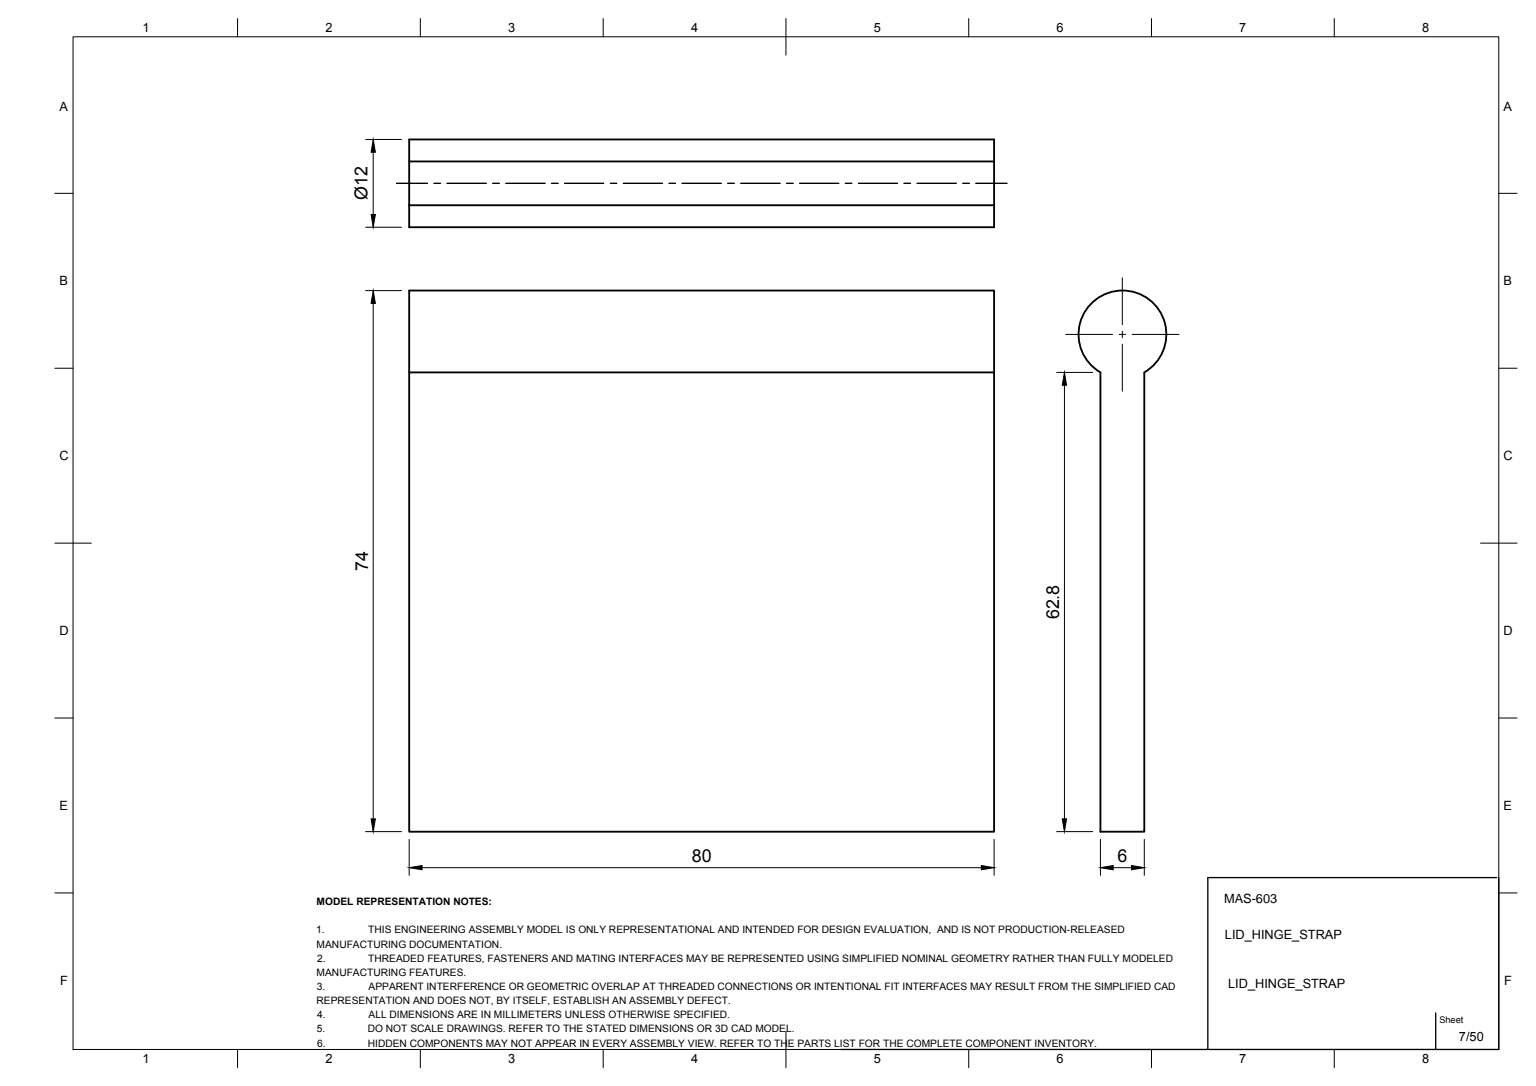
ISO-10303-21;
HEADER;
FILE_DESCRIPTION((''),'2;1');
FILE_NAME('LID_HINGE_STRAP.step','2026-10-01T22:06:14-07:00',(''),(''),'','','');
FILE_SCHEMA (('AUTOMOTIVE_DESIGN { 1 0 10303 214 3 1 1 }'));
ENDSEC;
DATA;
#10=MECHANICAL_DESIGN_GEOMETRIC_PRESENTATION_REPRESENTATION('',(#983),#50440);
#893=SHAPE_REPRESENTATION_RELATIONSHIP('SRR','None',#50623,#938) ;
#938=ADVANCED_BREP_SHAPE_REPRESENTATION('',(#1039),#50392) ;
#983=STYLED_ITEM('',(#50885),#1039) ;
#1039=MANIFOLD_SOLID_BREP('LID_HINGE_STRAP',#28631) ;
#1478=PLANE('',#29331) ;
#1479=PLANE('',#29332) ;
#1480=PLANE('',#29333) ;
#1481=PLANE('',#29334) ;
#1482=PLANE('',#29338) ;
#2419=FACE_OUTER_BOUND('',#3991,.T.) ;
#2420=FACE_OUTER_BOUND('',#3992,.T.) ;
#2421=FACE_OUTER_BOUND('',#3993,.T.) ;
#2422=FACE_OUTER_BOUND('',#3994,.T.) ;
#2423=FACE_OUTER_BOUND('',#3995,.T.) ;
#2424=FACE_OUTER_BOUND('',#3996,.T.) ;
#3991=EDGE_LOOP('',(#18977,#18978,#18979,#18980)) ;
#3992=EDGE_LOOP('',(#18981,#18982,#18983,#18984)) ;
#3993=EDGE_LOOP('',(#18985,#18986,#18987,#18988)) ;
#3994=EDGE_LOOP('',(#18989,#18990,#18991,#18992)) ;
#3995=EDGE_LOOP('',(#18993,#18994,#18995,#18996)) ;
#3996=EDGE_LOOP('',(#18997,#18998,#18999,#19000)) ;
#5885=LINE('',#41663,#8357) ;
#5886=LINE('',#41665,#8358) ;
#5887=LINE('',#41667,#8359) ;
#5888=LINE('',#41668,#8360) ;
#5889=LINE('',#41672,#8361) ;
#5890=LINE('',#41674,#8362) ;
#5891=LINE('',#41676,#8363) ;
#5892=LINE('',#41677,#8364) ;
#5893=LINE('',#41679,#8365) ;
#5894=LINE('',#41680,#8366) ;
#8357=VECTOR('',#32774,1.) ;
#8358=VECTOR('',#32775,1.) ;
#8359=VECTOR('',#32776,1.) ;
#8360=VECTOR('',#32777,1.) ;
#8361=VECTOR('',#32780,1.) ;
#8362=VECTOR('',#32781,1.) ;
#8363=VECTOR('',#32782,1.) ;
#8364=VECTOR('',#32783,1.) ;
#8365=VECTOR('',#32786,1.) ;
#8366=VECTOR('',#32787,1.) ;
#10724=CIRCLE('',#29335,0.6) ;
#10725=CIRCLE('',#29337,0.6) ;
#11983=VERTEX_POINT('',#41661) ;
#11984=VERTEX_POINT('',#41662) ;
#11985=VERTEX_POINT('',#41664) ;
#11986=VERTEX_POINT('',#41666) ;
#11987=VERTEX_POINT('',#41670) ;
#11988=VERTEX_POINT('',#41671) ;
#11989=VERTEX_POINT('',#41673) ;
#11990=VERTEX_POINT('',#41675) ;
#14754=EDGE_CURVE('',#11983,#11984,#5885,.T.) ;
#14755=EDGE_CURVE('',#11983,#11985,#5886,.T.) ;
#14756=EDGE_CURVE('',#11985,#11986,#5887,.T.) ;
#14757=EDGE_CURVE('',#11986,#11984,#5888,.T.) ;
#14758=EDGE_CURVE('',#11987,#11988,#5889,.T.) ;
#14759=EDGE_CURVE('',#11987,#11989,#5890,.T.) ;
#14760=EDGE_CURVE('',#11989,#11990,#5891,.T.) ;
#14761=EDGE_CURVE('',#11990,#11988,#5892,.T.) ;
#14762=EDGE_CURVE('',#11985,#11990,#5893,.T.) ;
#14763=EDGE_CURVE('',#11986,#11989,#5894,.T.) ;
#14764=EDGE_CURVE('',#11987,#11984,#10724,.T.) ;
#14765=EDGE_CURVE('',#11983,#11988,#10725,.T.) ;
#18977=ORIENTED_EDGE('',*,*,#14754,.F.) ;
#18978=ORIENTED_EDGE('',*,*,#14755,.T.) ;
#18979=ORIENTED_EDGE('',*,*,#14756,.T.) ;
#18980=ORIENTED_EDGE('',*,*,#14757,.T.) ;
#18981=ORIENTED_EDGE('',*,*,#14758,.F.) ;
#18982=ORIENTED_EDGE('',*,*,#14759,.T.) ;
#18983=ORIENTED_EDGE('',*,*,#14760,.T.) ;
#18984=ORIENTED_EDGE('',*,*,#14761,.T.) ;
#18985=ORIENTED_EDGE('',*,*,#14762,.T.) ;
#18986=ORIENTED_EDGE('',*,*,#14760,.F.) ;
#18987=ORIENTED_EDGE('',*,*,#14763,.F.) ;
#18988=ORIENTED_EDGE('',*,*,#14756,.F.) ;
#18989=ORIENTED_EDGE('',*,*,#14764,.T.) ;
#18990=ORIENTED_EDGE('',*,*,#14757,.F.) ;
#18991=ORIENTED_EDGE('',*,*,#14763,.T.) ;
#18992=ORIENTED_EDGE('',*,*,#14759,.F.) ;
#18993=ORIENTED_EDGE('',*,*,#14754,.T.) ;
#18994=ORIENTED_EDGE('',*,*,#14764,.F.) ;
#18995=ORIENTED_EDGE('',*,*,#14758,.T.) ;
#18996=ORIENTED_EDGE('',*,*,#14765,.F.) ;
#18997=ORIENTED_EDGE('',*,*,#14765,.T.) ;
#18998=ORIENTED_EDGE('',*,*,#14761,.F.) ;
#18999=ORIENTED_EDGE('',*,*,#14762,.F.) ;
#19000=ORIENTED_EDGE('',*,*,#14755,.F.) ;
#26658=CYLINDRICAL_SURFACE('',#29336,0.6) ;
#27154=ADVANCED_FACE('',(#2419),#1478,.T.) ;
#27155=ADVANCED_FACE('',(#2420),#1479,.F.) ;
#27156=ADVANCED_FACE('',(#2421),#1480,.F.) ;
#27157=ADVANCED_FACE('',(#2422),#1481,.T.) ;
#27158=ADVANCED_FACE('',(#2423),#26658,.T.) ;
#27159=ADVANCED_FACE('',(#2424),#1482,.T.) ;
#28631=CLOSED_SHELL('',(#27154,#27155,#27156,#27157,#27158,#27159)) ;
#29330=AXIS2_PLACEMENT_3D('',#41659,#32770,#32771) ;
#29331=AXIS2_PLACEMENT_3D('',#41660,#32772,#32773) ;
#29332=AXIS2_PLACEMENT_3D('',#41669,#32778,#32779) ;
#29333=AXIS2_PLACEMENT_3D('',#41678,#32784,#32785) ;
#29334=AXIS2_PLACEMENT_3D('',#41681,#32788,#32789) ;
#29335=AXIS2_PLACEMENT_3D('',#41682,#32790,#32791) ;
#29336=AXIS2_PLACEMENT_3D('',#41683,#32792,#32793) ;
#29337=AXIS2_PLACEMENT_3D('',#41684,#32794,#32795) ;
#29338=AXIS2_PLACEMENT_3D('',#41685,#32796,#32797) ;
#32770=DIRECTION('axis',(0.,0.,1.)) ;
#32771=DIRECTION('refdir',(1.,0.,0.)) ;
#32772=DIRECTION('center_axis',(0.,0.,1.)) ;
#32773=DIRECTION('ref_axis',(1.,0.,0.)) ;
#32774=DIRECTION('',(1.,0.,0.)) ;
#32775=DIRECTION('',(0.,-1.,0.)) ;
#32776=DIRECTION('',(1.,0.,0.)) ;
#32777=DIRECTION('',(0.,1.,0.)) ;
#32778=DIRECTION('center_axis',(0.,0.,1.)) ;
#32779=DIRECTION('ref_axis',(1.,0.,0.)) ;
#32780=DIRECTION('',(-1.,0.,0.)) ;
#32781=DIRECTION('',(0.,-1.,0.)) ;
#32782=DIRECTION('',(-1.,0.,0.)) ;
#32783=DIRECTION('',(0.,1.,0.)) ;
#32784=DIRECTION('center_axis',(0.,1.,0.)) ;
#32785=DIRECTION('ref_axis',(0.,0.,1.)) ;
#32786=DIRECTION('',(0.,0.,-1.)) ;
#32787=DIRECTION('',(0.,0.,-1.)) ;
#32788=DIRECTION('center_axis',(1.,0.,0.)) ;
#32789=DIRECTION('ref_axis',(0.,0.,-1.)) ;
#32790=DIRECTION('center_axis',(1.,0.,0.)) ;
#32791=DIRECTION('ref_axis',(0.,0.,-1.)) ;
#32792=DIRECTION('center_axis',(1.,0.,0.)) ;
#32793=DIRECTION('ref_axis',(0.,1.,1.83697019872103E-16)) ;
#32794=DIRECTION('center_axis',(-1.,0.,0.)) ;
#32795=DIRECTION('ref_axis',(0.,0.,-1.)) ;
#32796=DIRECTION('center_axis',(-1.,0.,0.)) ;
#32797=DIRECTION('ref_axis',(0.,0.,1.)) ;
#41659=CARTESIAN_POINT('',(0.,0.,0.)) ;
#41660=CARTESIAN_POINT('Origin',(0.,53.4,112.6)) ;
#41661=CARTESIAN_POINT('',(-4.,56.2803847577293,112.6)) ;
#41662=CARTESIAN_POINT('',(4.,56.2803847577293,112.6)) ;
#41663=CARTESIAN_POINT('',(0.,56.2803847577293,112.6)) ;
#41664=CARTESIAN_POINT('',(-4.,50.,112.6)) ;
#41665=CARTESIAN_POINT('',(-4.,53.4,112.6)) ;
#41666=CARTESIAN_POINT('',(4.,50.,112.6)) ;
#41667=CARTESIAN_POINT('',(0.,50.,112.6)) ;
#41668=CARTESIAN_POINT('',(4.,53.4,112.6)) ;
#41669=CARTESIAN_POINT('Origin',(0.,53.4,112.)) ;
#41670=CARTESIAN_POINT('',(4.,56.2803847577293,112.)) ;
#41671=CARTESIAN_POINT('',(-4.,56.2803847577293,112.)) ;
#41672=CARTESIAN_POINT('',(0.,56.2803847577293,112.)) ;
#41673=CARTESIAN_POINT('',(4.,50.,112.)) ;
#41674=CARTESIAN_POINT('',(4.,53.4,112.)) ;
#41675=CARTESIAN_POINT('',(-4.,50.,112.)) ;
#41676=CARTESIAN_POINT('',(0.,50.,112.)) ;
#41677=CARTESIAN_POINT('',(-4.,53.4,112.)) ;
#41678=CARTESIAN_POINT('Origin',(0.,50.,112.3)) ;
#41679=CARTESIAN_POINT('',(-4.,50.,112.3)) ;
#41680=CARTESIAN_POINT('',(4.,50.,112.3)) ;
#41681=CARTESIAN_POINT('Origin',(4.,56.8,112.3)) ;
#41682=CARTESIAN_POINT('Origin',(4.,56.8,112.3)) ;
#41683=CARTESIAN_POINT('Origin',(0.,56.8,112.3)) ;
#41684=CARTESIAN_POINT('Origin',(-4.,56.8,112.3)) ;
#41685=CARTESIAN_POINT('Origin',(-4.,56.8,112.3)) ;
#50339=UNCERTAINTY_MEASURE_WITH_UNIT(LENGTH_MEASURE(0.001),#50441,
'DISTANCE_ACCURACY_VALUE',
'Maximum model space distance between geometric entities at asserted c
onnectivities') ;
#50387=UNCERTAINTY_MEASURE_WITH_UNIT(LENGTH_MEASURE(0.001),#50441,
'DISTANCE_ACCURACY_VALUE',
'Maximum model space distance between geometric entities at asserted c
onnectivities') ;
#50392=(
GEOMETRIC_REPRESENTATION_CONTEXT(3)
GLOBAL_UNCERTAINTY_ASSIGNED_CONTEXT((#50339))
GLOBAL_UNIT_ASSIGNED_CONTEXT((#50441,#50443,#50444))
REPRESENTATION_CONTEXT('','3D')
) ;
#50440=(
GEOMETRIC_REPRESENTATION_CONTEXT(3)
GLOBAL_UNCERTAINTY_ASSIGNED_CONTEXT((#50387))
GLOBAL_UNIT_ASSIGNED_CONTEXT((#50441,#50443,#50444))
REPRESENTATION_CONTEXT('','3D')
) ;
#50441=(
LENGTH_UNIT()
NAMED_UNIT(*)
SI_UNIT(.CENTI.,.METRE.)
) ;
#50443=(
NAMED_UNIT(*)
PLANE_ANGLE_UNIT()
SI_UNIT($,.RADIAN.)
) ;
#50444=(
NAMED_UNIT(*)
SI_UNIT($,.STERADIAN.)
SOLID_ANGLE_UNIT()
) ;
#50449=SHAPE_DEFINITION_REPRESENTATION(#50501,#50623) ;
#50501=PRODUCT_DEFINITION_SHAPE('',$,#50676) ;
#50623=SHAPE_REPRESENTATION('',(#29330),#50392) ;
#50671=PRODUCT_DEFINITION_CONTEXT('part definition',#50829,'design') ;
#50676=PRODUCT_DEFINITION('LID_HINGE_STRAP','LID_HINGE_STRAP',#50728,
#50671) ;
#50728=PRODUCT_DEFINITION_FORMATION('',$,#50835) ;
#50829=APPLICATION_CONTEXT(
'Core Data for Automotive Mechanical Design Process') ;
#50830=PRODUCT_CONTEXT('part definition',#50829,'mechanical') ;
#50835=PRODUCT('LID_HINGE_STRAP','LID_HINGE_STRAP',$,(#50830)) ;
#50885=PRESENTATION_STYLE_ASSIGNMENT((#50892)) ;
#50892=SURFACE_STYLE_USAGE(.BOTH.,#50899) ;
#50899=SURFACE_SIDE_STYLE('',(#50906)) ;
#50906=SURFACE_STYLE_FILL_AREA(#50913) ;
#50913=FILL_AREA_STYLE('Steel - Galvanized (Small)',(#50920)) ;
#50920=FILL_AREA_STYLE_COLOUR('Steel - Galvanized (Small)',#50927) ;
#50927=COLOUR_RGB('Steel - Galvanized (Small)', 0.09019608, 0.27058824, 0.51372549) ;
ENDSEC;
END-ISO-10303-21;
